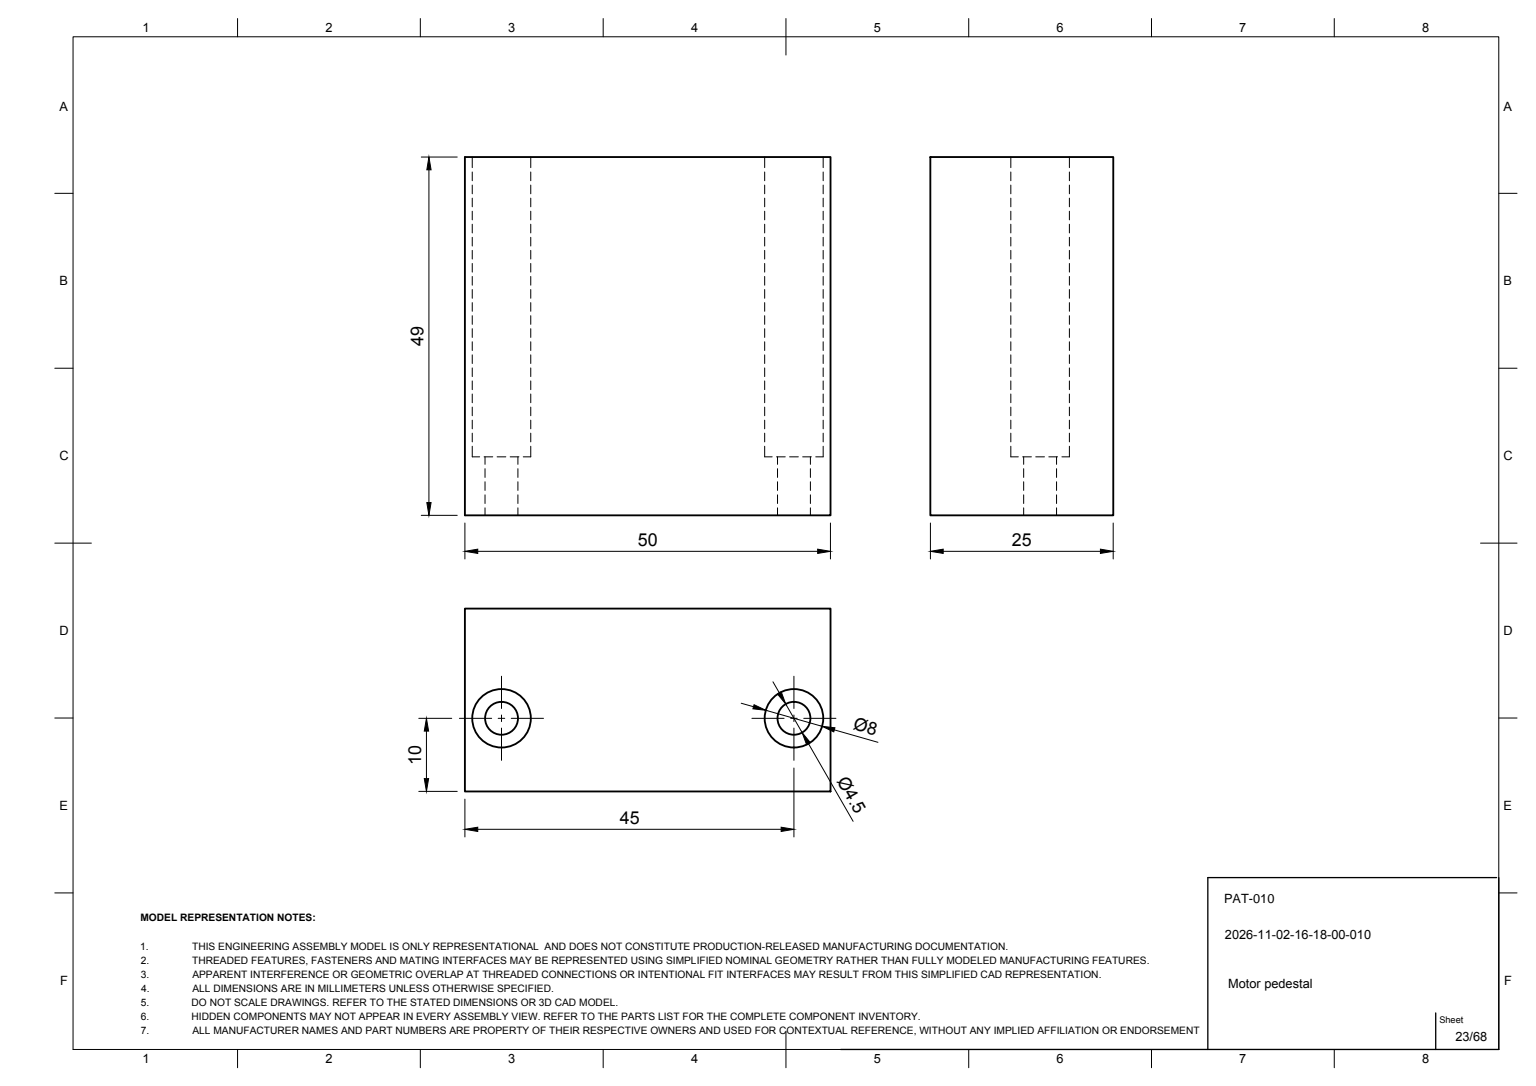
ISO-10303-21;
HEADER;
/* Generated by software containing ST-Developer
 * from STEP Tools, Inc. (www.steptools.com) 
 */

FILE_DESCRIPTION(
/* description */ ('Belt conveyor head drive unit'),
/* implementation_level */ '2;1');

FILE_NAME(
/* name */ 'Motor pedestal.step',
/* time_stamp */ '2026-10-28T03:26:19-07:00',
/* author */ (''),
/* organization */ (''),
/* preprocessor_version */ 'ST-DEVELOPER v20.2',
/* originating_system */ 'Autodesk Translation Framework v15.17.0.0',
/* authorisation */ '');

FILE_SCHEMA (('AUTOMOTIVE_DESIGN { 1 0 10303 214 3 1 1 }'));
ENDSEC;

DATA;
#10=MECHANICAL_DESIGN_GEOMETRIC_PRESENTATION_REPRESENTATION('',(#869),#27069);
#731=SHAPE_REPRESENTATION_RELATIONSHIP('SRR','None',#27375,#800);
#800=ADVANCED_BREP_SHAPE_REPRESENTATION('',(#954),#27017);
#869=STYLED_ITEM('',(#27783),#954);
#954=MANIFOLD_SOLID_BREP('Body1',#13734);
#1129=FACE_BOUND('',#2810,.T.);
#1130=FACE_BOUND('',#2814,.T.);
#1131=FACE_BOUND('',#2821,.T.);
#1132=FACE_BOUND('',#2822,.T.);
#1133=FACE_BOUND('',#2824,.T.);
#1134=FACE_BOUND('',#2825,.T.);
#1405=PLANE('',#15120);
#1406=PLANE('',#15127);
#1407=PLANE('',#15131);
#1408=PLANE('',#15132);
#1409=PLANE('',#15133);
#1410=PLANE('',#15134);
#1411=PLANE('',#15135);
#1412=PLANE('',#15136);
#1891=FACE_OUTER_BOUND('',#2808,.T.);
#1892=FACE_OUTER_BOUND('',#2809,.T.);
#1893=FACE_OUTER_BOUND('',#2811,.T.);
#1894=FACE_OUTER_BOUND('',#2812,.T.);
#1895=FACE_OUTER_BOUND('',#2813,.T.);
#1896=FACE_OUTER_BOUND('',#2815,.T.);
#1897=FACE_OUTER_BOUND('',#2816,.T.);
#1898=FACE_OUTER_BOUND('',#2817,.T.);
#1899=FACE_OUTER_BOUND('',#2818,.T.);
#1900=FACE_OUTER_BOUND('',#2819,.T.);
#1901=FACE_OUTER_BOUND('',#2820,.T.);
#1902=FACE_OUTER_BOUND('',#2823,.T.);
#2808=EDGE_LOOP('',(#10080,#10081,#10082,#10083));
#2809=EDGE_LOOP('',(#10084));
#2810=EDGE_LOOP('',(#10085));
#2811=EDGE_LOOP('',(#10086,#10087,#10088,#10089));
#2812=EDGE_LOOP('',(#10090,#10091,#10092,#10093));
#2813=EDGE_LOOP('',(#10094));
#2814=EDGE_LOOP('',(#10095));
#2815=EDGE_LOOP('',(#10096,#10097,#10098,#10099));
#2816=EDGE_LOOP('',(#10100,#10101,#10102,#10103));
#2817=EDGE_LOOP('',(#10104,#10105,#10106,#10107));
#2818=EDGE_LOOP('',(#10108,#10109,#10110,#10111));
#2819=EDGE_LOOP('',(#10112,#10113,#10114,#10115));
#2820=EDGE_LOOP('',(#10116,#10117,#10118,#10119));
#2821=EDGE_LOOP('',(#10120));
#2822=EDGE_LOOP('',(#10121));
#2823=EDGE_LOOP('',(#10122,#10123,#10124,#10125));
#2824=EDGE_LOOP('',(#10126));
#2825=EDGE_LOOP('',(#10127));
#3787=LINE('',#22192,#4579);
#3788=LINE('',#22200,#4580);
#3789=LINE('',#22205,#4581);
#3790=LINE('',#22213,#4582);
#3791=LINE('',#22217,#4583);
#3792=LINE('',#22219,#4584);
#3793=LINE('',#22221,#4585);
#3794=LINE('',#22222,#4586);
#3795=LINE('',#22225,#4587);
#3796=LINE('',#22227,#4588);
#3797=LINE('',#22228,#4589);
#3798=LINE('',#22231,#4590);
#3799=LINE('',#22233,#4591);
#3800=LINE('',#22234,#4592);
#3801=LINE('',#22236,#4593);
#3802=LINE('',#22237,#4594);
#4579=VECTOR('',#17837,0.4);
#4580=VECTOR('',#17848,0.225);
#4581=VECTOR('',#17853,0.4);
#4582=VECTOR('',#17864,0.225);
#4583=VECTOR('',#17867,1.);
#4584=VECTOR('',#17868,1.);
#4585=VECTOR('',#17869,1.);
#4586=VECTOR('',#17870,1.);
#4587=VECTOR('',#17873,1.);
#4588=VECTOR('',#17874,1.);
#4589=VECTOR('',#17875,1.);
#4590=VECTOR('',#17878,1.);
#4591=VECTOR('',#17879,1.);
#4592=VECTOR('',#17880,1.);
#4593=VECTOR('',#17883,1.);
#4594=VECTOR('',#17884,1.);
#5354=CIRCLE('',#15118,0.4);
#5355=CIRCLE('',#15119,0.4);
#5356=CIRCLE('',#15121,0.225);
#5357=CIRCLE('',#15123,0.225);
#5358=CIRCLE('',#15125,0.4);
#5359=CIRCLE('',#15126,0.4);
#5360=CIRCLE('',#15128,0.225);
#5361=CIRCLE('',#15130,0.225);
#6327=VERTEX_POINT('',#22189);
#6328=VERTEX_POINT('',#22191);
#6329=VERTEX_POINT('',#22195);
#6330=VERTEX_POINT('',#22198);
#6331=VERTEX_POINT('',#22202);
#6332=VERTEX_POINT('',#22204);
#6333=VERTEX_POINT('',#22208);
#6334=VERTEX_POINT('',#22211);
#6335=VERTEX_POINT('',#22215);
#6336=VERTEX_POINT('',#22216);
#6337=VERTEX_POINT('',#22218);
#6338=VERTEX_POINT('',#22220);
#6339=VERTEX_POINT('',#22224);
#6340=VERTEX_POINT('',#22226);
#6341=VERTEX_POINT('',#22230);
#6342=VERTEX_POINT('',#22232);
#7732=EDGE_CURVE('',#6327,#6327,#5354,.T.);
#7733=EDGE_CURVE('',#6327,#6328,#3787,.T.);
#7734=EDGE_CURVE('',#6328,#6328,#5355,.T.);
#7735=EDGE_CURVE('',#6329,#6329,#5356,.T.);
#7736=EDGE_CURVE('',#6330,#6330,#5357,.T.);
#7737=EDGE_CURVE('',#6330,#6329,#3788,.T.);
#7738=EDGE_CURVE('',#6331,#6331,#5358,.T.);
#7739=EDGE_CURVE('',#6331,#6332,#3789,.T.);
#7740=EDGE_CURVE('',#6332,#6332,#5359,.T.);
#7741=EDGE_CURVE('',#6333,#6333,#5360,.T.);
#7742=EDGE_CURVE('',#6334,#6334,#5361,.T.);
#7743=EDGE_CURVE('',#6334,#6333,#3790,.T.);
#7744=EDGE_CURVE('',#6335,#6336,#3791,.T.);
#7745=EDGE_CURVE('',#6336,#6337,#3792,.T.);
#7746=EDGE_CURVE('',#6338,#6337,#3793,.T.);
#7747=EDGE_CURVE('',#6335,#6338,#3794,.T.);
#7748=EDGE_CURVE('',#6339,#6335,#3795,.T.);
#7749=EDGE_CURVE('',#6340,#6338,#3796,.T.);
#7750=EDGE_CURVE('',#6339,#6340,#3797,.T.);
#7751=EDGE_CURVE('',#6341,#6339,#3798,.T.);
#7752=EDGE_CURVE('',#6342,#6340,#3799,.T.);
#7753=EDGE_CURVE('',#6341,#6342,#3800,.T.);
#7754=EDGE_CURVE('',#6336,#6341,#3801,.T.);
#7755=EDGE_CURVE('',#6337,#6342,#3802,.T.);
#10080=ORIENTED_EDGE('',*,*,#7732,.F.);
#10081=ORIENTED_EDGE('',*,*,#7733,.T.);
#10082=ORIENTED_EDGE('',*,*,#7734,.F.);
#10083=ORIENTED_EDGE('',*,*,#7733,.F.);
#10084=ORIENTED_EDGE('',*,*,#7732,.T.);
#10085=ORIENTED_EDGE('',*,*,#7735,.F.);
#10086=ORIENTED_EDGE('',*,*,#7736,.F.);
#10087=ORIENTED_EDGE('',*,*,#7737,.T.);
#10088=ORIENTED_EDGE('',*,*,#7735,.T.);
#10089=ORIENTED_EDGE('',*,*,#7737,.F.);
#10090=ORIENTED_EDGE('',*,*,#7738,.F.);
#10091=ORIENTED_EDGE('',*,*,#7739,.T.);
#10092=ORIENTED_EDGE('',*,*,#7740,.F.);
#10093=ORIENTED_EDGE('',*,*,#7739,.F.);
#10094=ORIENTED_EDGE('',*,*,#7738,.T.);
#10095=ORIENTED_EDGE('',*,*,#7741,.F.);
#10096=ORIENTED_EDGE('',*,*,#7742,.F.);
#10097=ORIENTED_EDGE('',*,*,#7743,.T.);
#10098=ORIENTED_EDGE('',*,*,#7741,.T.);
#10099=ORIENTED_EDGE('',*,*,#7743,.F.);
#10100=ORIENTED_EDGE('',*,*,#7744,.T.);
#10101=ORIENTED_EDGE('',*,*,#7745,.T.);
#10102=ORIENTED_EDGE('',*,*,#7746,.F.);
#10103=ORIENTED_EDGE('',*,*,#7747,.F.);
#10104=ORIENTED_EDGE('',*,*,#7748,.T.);
#10105=ORIENTED_EDGE('',*,*,#7747,.T.);
#10106=ORIENTED_EDGE('',*,*,#7749,.F.);
#10107=ORIENTED_EDGE('',*,*,#7750,.F.);
#10108=ORIENTED_EDGE('',*,*,#7751,.T.);
#10109=ORIENTED_EDGE('',*,*,#7750,.T.);
#10110=ORIENTED_EDGE('',*,*,#7752,.F.);
#10111=ORIENTED_EDGE('',*,*,#7753,.F.);
#10112=ORIENTED_EDGE('',*,*,#7754,.T.);
#10113=ORIENTED_EDGE('',*,*,#7753,.T.);
#10114=ORIENTED_EDGE('',*,*,#7755,.F.);
#10115=ORIENTED_EDGE('',*,*,#7745,.F.);
#10116=ORIENTED_EDGE('',*,*,#7755,.T.);
#10117=ORIENTED_EDGE('',*,*,#7752,.T.);
#10118=ORIENTED_EDGE('',*,*,#7749,.T.);
#10119=ORIENTED_EDGE('',*,*,#7746,.T.);
#10120=ORIENTED_EDGE('',*,*,#7734,.T.);
#10121=ORIENTED_EDGE('',*,*,#7740,.T.);
#10122=ORIENTED_EDGE('',*,*,#7754,.F.);
#10123=ORIENTED_EDGE('',*,*,#7744,.F.);
#10124=ORIENTED_EDGE('',*,*,#7748,.F.);
#10125=ORIENTED_EDGE('',*,*,#7751,.F.);
#10126=ORIENTED_EDGE('',*,*,#7736,.T.);
#10127=ORIENTED_EDGE('',*,*,#7742,.T.);
#12662=CYLINDRICAL_SURFACE('',#15117,0.4);
#12663=CYLINDRICAL_SURFACE('',#15122,0.225);
#12664=CYLINDRICAL_SURFACE('',#15124,0.4);
#12665=CYLINDRICAL_SURFACE('',#15129,0.225);
#13170=ADVANCED_FACE('',(#1891),#12662,.F.);
#13171=ADVANCED_FACE('',(#1892,#1129),#1405,.T.);
#13172=ADVANCED_FACE('',(#1893),#12663,.F.);
#13173=ADVANCED_FACE('',(#1894),#12664,.F.);
#13174=ADVANCED_FACE('',(#1895,#1130),#1406,.T.);
#13175=ADVANCED_FACE('',(#1896),#12665,.F.);
#13176=ADVANCED_FACE('',(#1897),#1407,.T.);
#13177=ADVANCED_FACE('',(#1898),#1408,.T.);
#13178=ADVANCED_FACE('',(#1899),#1409,.T.);
#13179=ADVANCED_FACE('',(#1900),#1410,.T.);
#13180=ADVANCED_FACE('',(#1901,#1131,#1132),#1411,.T.);
#13181=ADVANCED_FACE('',(#1902,#1133,#1134),#1412,.F.);
#13734=CLOSED_SHELL('',(#13170,#13171,#13172,#13173,#13174,#13175,#13176,
#13177,#13178,#13179,#13180,#13181));
#15116=AXIS2_PLACEMENT_3D('',#22187,#17831,#17832);
#15117=AXIS2_PLACEMENT_3D('',#22188,#17833,#17834);
#15118=AXIS2_PLACEMENT_3D('',#22190,#17835,#17836);
#15119=AXIS2_PLACEMENT_3D('',#22193,#17838,#17839);
#15120=AXIS2_PLACEMENT_3D('',#22194,#17840,#17841);
#15121=AXIS2_PLACEMENT_3D('',#22196,#17842,#17843);
#15122=AXIS2_PLACEMENT_3D('',#22197,#17844,#17845);
#15123=AXIS2_PLACEMENT_3D('',#22199,#17846,#17847);
#15124=AXIS2_PLACEMENT_3D('',#22201,#17849,#17850);
#15125=AXIS2_PLACEMENT_3D('',#22203,#17851,#17852);
#15126=AXIS2_PLACEMENT_3D('',#22206,#17854,#17855);
#15127=AXIS2_PLACEMENT_3D('',#22207,#17856,#17857);
#15128=AXIS2_PLACEMENT_3D('',#22209,#17858,#17859);
#15129=AXIS2_PLACEMENT_3D('',#22210,#17860,#17861);
#15130=AXIS2_PLACEMENT_3D('',#22212,#17862,#17863);
#15131=AXIS2_PLACEMENT_3D('',#22214,#17865,#17866);
#15132=AXIS2_PLACEMENT_3D('',#22223,#17871,#17872);
#15133=AXIS2_PLACEMENT_3D('',#22229,#17876,#17877);
#15134=AXIS2_PLACEMENT_3D('',#22235,#17881,#17882);
#15135=AXIS2_PLACEMENT_3D('',#22238,#17885,#17886);
#15136=AXIS2_PLACEMENT_3D('',#22239,#17887,#17888);
#17831=DIRECTION('axis',(0.,0.,1.));
#17832=DIRECTION('refdir',(1.,0.,0.));
#17833=DIRECTION('center_axis',(0.,0.,1.));
#17834=DIRECTION('ref_axis',(1.,0.,0.));
#17835=DIRECTION('center_axis',(0.,0.,1.));
#17836=DIRECTION('ref_axis',(1.,0.,0.));
#17837=DIRECTION('',(0.,0.,1.));
#17838=DIRECTION('center_axis',(0.,0.,-1.));
#17839=DIRECTION('ref_axis',(1.,0.,0.));
#17840=DIRECTION('center_axis',(0.,0.,1.));
#17841=DIRECTION('ref_axis',(1.,0.,0.));
#17842=DIRECTION('center_axis',(0.,0.,1.));
#17843=DIRECTION('ref_axis',(1.,0.,0.));
#17844=DIRECTION('center_axis',(0.,0.,1.));
#17845=DIRECTION('ref_axis',(1.,0.,0.));
#17846=DIRECTION('center_axis',(0.,0.,1.));
#17847=DIRECTION('ref_axis',(1.,0.,0.));
#17848=DIRECTION('',(0.,0.,1.));
#17849=DIRECTION('center_axis',(0.,0.,1.));
#17850=DIRECTION('ref_axis',(1.,0.,0.));
#17851=DIRECTION('center_axis',(0.,0.,1.));
#17852=DIRECTION('ref_axis',(1.,0.,0.));
#17853=DIRECTION('',(0.,0.,1.));
#17854=DIRECTION('center_axis',(0.,0.,-1.));
#17855=DIRECTION('ref_axis',(1.,0.,0.));
#17856=DIRECTION('center_axis',(0.,0.,1.));
#17857=DIRECTION('ref_axis',(1.,0.,0.));
#17858=DIRECTION('center_axis',(0.,0.,1.));
#17859=DIRECTION('ref_axis',(1.,0.,0.));
#17860=DIRECTION('center_axis',(0.,0.,1.));
#17861=DIRECTION('ref_axis',(1.,0.,0.));
#17862=DIRECTION('center_axis',(0.,0.,1.));
#17863=DIRECTION('ref_axis',(1.,0.,0.));
#17864=DIRECTION('',(0.,0.,1.));
#17865=DIRECTION('center_axis',(0.,1.,0.));
#17866=DIRECTION('ref_axis',(-1.,0.,0.));
#17867=DIRECTION('',(-1.,0.,0.));
#17868=DIRECTION('',(0.,0.,1.));
#17869=DIRECTION('',(-1.,0.,0.));
#17870=DIRECTION('',(0.,0.,1.));
#17871=DIRECTION('center_axis',(1.,0.,0.));
#17872=DIRECTION('ref_axis',(0.,1.,0.));
#17873=DIRECTION('',(0.,1.,0.));
#17874=DIRECTION('',(0.,1.,0.));
#17875=DIRECTION('',(0.,0.,1.));
#17876=DIRECTION('center_axis',(0.,-1.,0.));
#17877=DIRECTION('ref_axis',(1.,0.,0.));
#17878=DIRECTION('',(1.,0.,0.));
#17879=DIRECTION('',(1.,0.,0.));
#17880=DIRECTION('',(0.,0.,1.));
#17881=DIRECTION('center_axis',(-1.,0.,0.));
#17882=DIRECTION('ref_axis',(0.,-1.,0.));
#17883=DIRECTION('',(0.,-1.,0.));
#17884=DIRECTION('',(0.,-1.,0.));
#17885=DIRECTION('center_axis',(0.,0.,1.));
#17886=DIRECTION('ref_axis',(1.,0.,0.));
#17887=DIRECTION('center_axis',(0.,0.,1.));
#17888=DIRECTION('ref_axis',(1.,0.,0.));
#22187=CARTESIAN_POINT('',(0.,0.,0.));
#22188=CARTESIAN_POINT('Origin',(-1.5,8.5,0.8));
#22189=CARTESIAN_POINT('',(-1.9,8.5,0.8));
#22190=CARTESIAN_POINT('Origin',(-1.5,8.5,0.8));
#22191=CARTESIAN_POINT('',(-1.9,8.5,4.9));
#22192=CARTESIAN_POINT('',(-1.9,8.5,0.8));
#22193=CARTESIAN_POINT('Origin',(-1.5,8.5,4.9));
#22194=CARTESIAN_POINT('Origin',(-1.5,8.5,0.8));
#22195=CARTESIAN_POINT('',(-1.725,8.5,0.8));
#22196=CARTESIAN_POINT('Origin',(-1.5,8.5,0.8));
#22197=CARTESIAN_POINT('Origin',(-1.5,8.5,-0.1));
#22198=CARTESIAN_POINT('',(-1.725,8.5,0.));
#22199=CARTESIAN_POINT('Origin',(-1.5,8.5,0.));
#22200=CARTESIAN_POINT('',(-1.725,8.5,-0.1));
#22201=CARTESIAN_POINT('Origin',(-1.5,4.5,0.8));
#22202=CARTESIAN_POINT('',(-1.9,4.5,0.8));
#22203=CARTESIAN_POINT('Origin',(-1.5,4.5,0.8));
#22204=CARTESIAN_POINT('',(-1.9,4.5,4.9));
#22205=CARTESIAN_POINT('',(-1.9,4.5,0.8));
#22206=CARTESIAN_POINT('Origin',(-1.5,4.5,4.9));
#22207=CARTESIAN_POINT('Origin',(-1.5,4.5,0.8));
#22208=CARTESIAN_POINT('',(-1.725,4.5,0.8));
#22209=CARTESIAN_POINT('Origin',(-1.5,4.5,0.8));
#22210=CARTESIAN_POINT('Origin',(-1.5,4.5,-0.1));
#22211=CARTESIAN_POINT('',(-1.725,4.5,0.));
#22212=CARTESIAN_POINT('Origin',(-1.5,4.5,0.));
#22213=CARTESIAN_POINT('',(-1.725,4.5,-0.1));
#22214=CARTESIAN_POINT('Origin',(0.,9.,0.));
#22215=CARTESIAN_POINT('',(0.,9.,0.));
#22216=CARTESIAN_POINT('',(-2.5,9.,0.));
#22217=CARTESIAN_POINT('',(0.,9.,0.));
#22218=CARTESIAN_POINT('',(-2.5,9.,4.9));
#22219=CARTESIAN_POINT('',(-2.5,9.,0.));
#22220=CARTESIAN_POINT('',(0.,9.,4.9));
#22221=CARTESIAN_POINT('',(0.,9.,4.9));
#22222=CARTESIAN_POINT('',(0.,9.,0.));
#22223=CARTESIAN_POINT('Origin',(0.,4.,0.));
#22224=CARTESIAN_POINT('',(0.,4.,0.));
#22225=CARTESIAN_POINT('',(0.,4.,0.));
#22226=CARTESIAN_POINT('',(0.,4.,4.9));
#22227=CARTESIAN_POINT('',(0.,4.,4.9));
#22228=CARTESIAN_POINT('',(0.,4.,0.));
#22229=CARTESIAN_POINT('Origin',(-2.5,4.,0.));
#22230=CARTESIAN_POINT('',(-2.5,4.,0.));
#22231=CARTESIAN_POINT('',(-2.5,4.,0.));
#22232=CARTESIAN_POINT('',(-2.5,4.,4.9));
#22233=CARTESIAN_POINT('',(-2.5,4.,4.9));
#22234=CARTESIAN_POINT('',(-2.5,4.,0.));
#22235=CARTESIAN_POINT('Origin',(-2.5,9.,0.));
#22236=CARTESIAN_POINT('',(-2.5,9.,0.));
#22237=CARTESIAN_POINT('',(-2.5,9.,4.9));
#22238=CARTESIAN_POINT('Origin',(-1.25,6.5,4.9));
#22239=CARTESIAN_POINT('Origin',(-1.25,6.5,0.));
#26940=UNCERTAINTY_MEASURE_WITH_UNIT(LENGTH_MEASURE(0.001),#27070,
'DISTANCE_ACCURACY_VALUE',
'Maximum model space distance between geometric entities at asserted c
onnectivities');
#26992=UNCERTAINTY_MEASURE_WITH_UNIT(LENGTH_MEASURE(0.001),#27070,
'DISTANCE_ACCURACY_VALUE',
'Maximum model space distance between geometric entities at asserted c
onnectivities');
#27017=(
GEOMETRIC_REPRESENTATION_CONTEXT(3)
GLOBAL_UNCERTAINTY_ASSIGNED_CONTEXT((#26940))
GLOBAL_UNIT_ASSIGNED_CONTEXT((#27070,#27072,#27073))
REPRESENTATION_CONTEXT('','3D')
);
#27069=(
GEOMETRIC_REPRESENTATION_CONTEXT(3)
GLOBAL_UNCERTAINTY_ASSIGNED_CONTEXT((#26992))
GLOBAL_UNIT_ASSIGNED_CONTEXT((#27070,#27072,#27073))
REPRESENTATION_CONTEXT('','3D')
);
#27070=(
LENGTH_UNIT()
NAMED_UNIT(*)
SI_UNIT(.CENTI.,.METRE.)
);
#27072=(
NAMED_UNIT(*)
PLANE_ANGLE_UNIT()
SI_UNIT($,.RADIAN.)
);
#27073=(
NAMED_UNIT(*)
SI_UNIT($,.STERADIAN.)
SOLID_ANGLE_UNIT()
);
#27098=SHAPE_DEFINITION_REPRESENTATION(#27174,#27375);
#27174=PRODUCT_DEFINITION_SHAPE('',$,#27452);
#27375=SHAPE_REPRESENTATION('',(#15116),#27017);
#27427=PRODUCT_DEFINITION_CONTEXT('part definition',#27657,'design');
#27452=PRODUCT_DEFINITION('Motor pedestal','Motor pedestal',#27528,#27427);
#27528=PRODUCT_DEFINITION_FORMATION('',$,#27683);
#27657=APPLICATION_CONTEXT(
'Core Data for Automotive Mechanical Design Process');
#27658=PRODUCT_CONTEXT('part definition',#27657,'mechanical');
#27683=PRODUCT('Motor pedestal','Motor pedestal','Motor pedestal',(#27658));
#27777=COLOUR_RGB('Light Blue',0.38,0.62,0.78);
#27778=FILL_AREA_STYLE_COLOUR('',#27777);
#27779=FILL_AREA_STYLE('',(#27778));
#27780=SURFACE_STYLE_FILL_AREA(#27779);
#27781=SURFACE_SIDE_STYLE('',(#27780));
#27782=SURFACE_STYLE_USAGE(.BOTH.,#27781);
#27783=PRESENTATION_STYLE_ASSIGNMENT((#27782));
ENDSEC;
END-ISO-10303-21;
